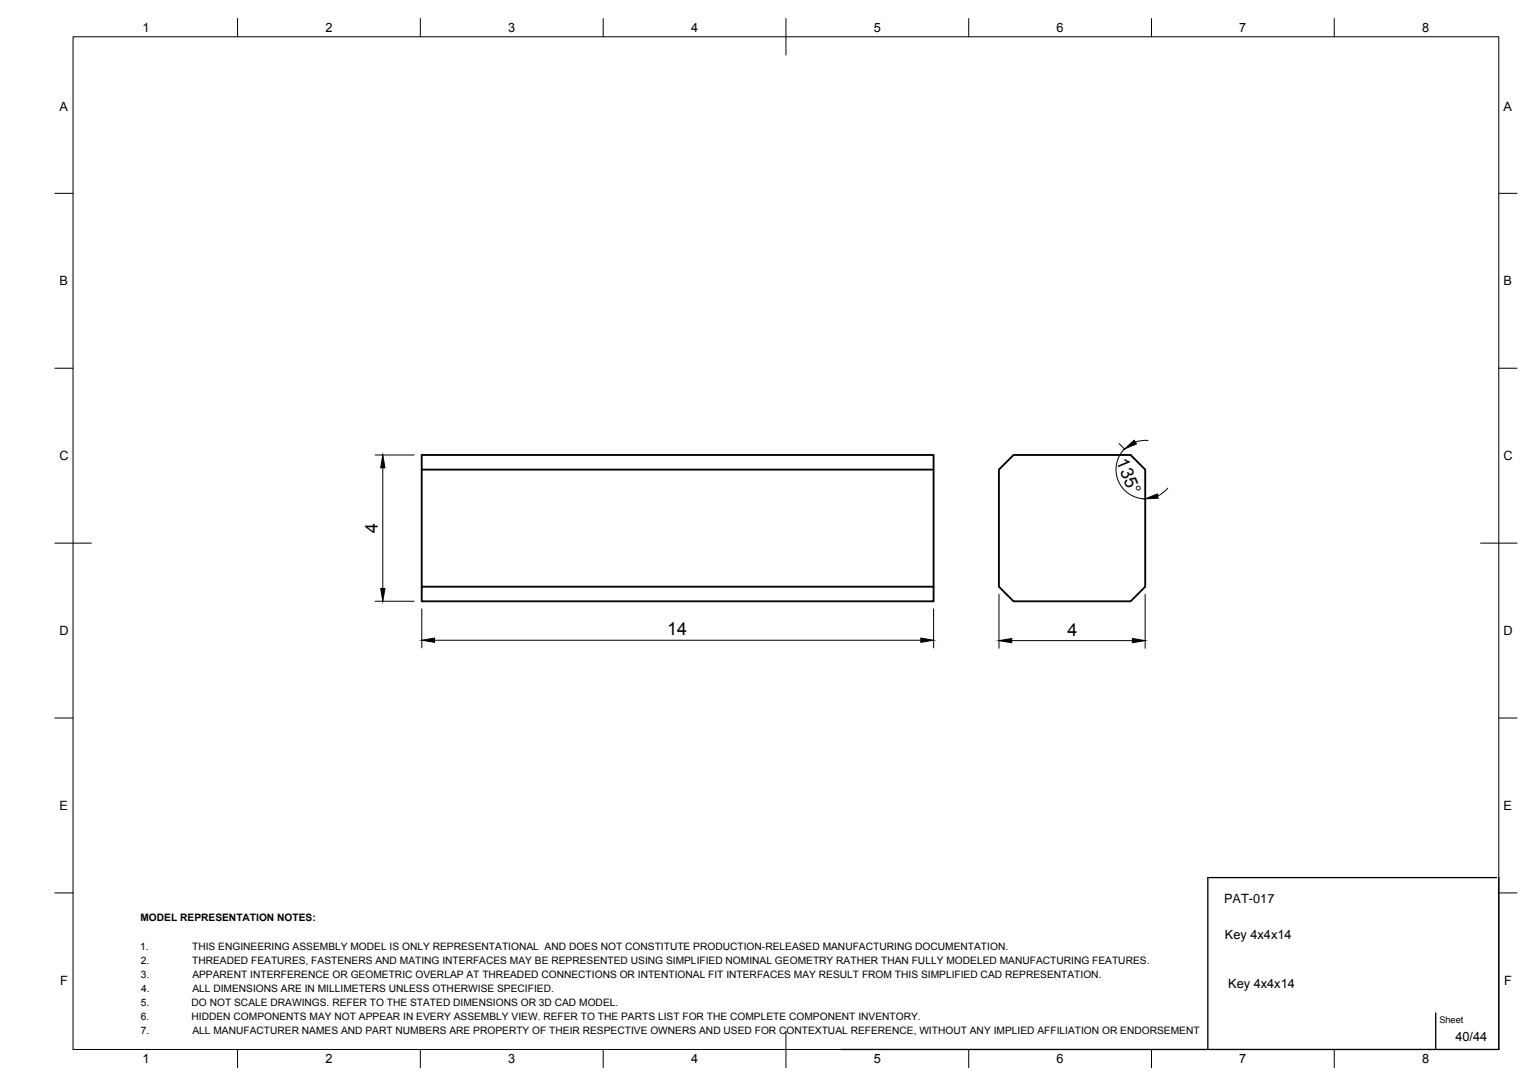
ISO-10303-21;
HEADER;
/* Generated by software containing ST-Developer
 * from STEP Tools, Inc. (www.steptools.com) 
 */

FILE_DESCRIPTION(
/* description */ ('Cam-and-follower valve demonstrator'),
/* implementation_level */ '2;1');

FILE_NAME(
/* name */ 'Key 4x4x14.step',
/* time_stamp */ '2026-10-28T03:25:17-07:00',
/* author */ (''),
/* organization */ (''),
/* preprocessor_version */ 'ST-DEVELOPER v20.2',
/* originating_system */ 'Autodesk Translation Framework v15.17.0.0',
/* authorisation */ '');

FILE_SCHEMA (('AUTOMOTIVE_DESIGN { 1 0 10303 214 3 1 1 }'));
ENDSEC;

DATA;
#10=MECHANICAL_DESIGN_GEOMETRIC_PRESENTATION_REPRESENTATION('',(#450),#12896);
#371=SHAPE_REPRESENTATION_RELATIONSHIP('SRR','None',#13090,#407);
#407=ADVANCED_BREP_SHAPE_REPRESENTATION('',(#491),#12890);
#450=STYLED_ITEM('',(#13330),#491);
#491=MANIFOLD_SOLID_BREP('Body1',#6219);
#1418=FACE_OUTER_BOUND('',#1943,.T.);
#1419=FACE_OUTER_BOUND('',#1944,.T.);
#1420=FACE_OUTER_BOUND('',#1945,.T.);
#1421=FACE_OUTER_BOUND('',#1946,.T.);
#1422=FACE_OUTER_BOUND('',#1947,.T.);
#1423=FACE_OUTER_BOUND('',#1948,.T.);
#1424=FACE_OUTER_BOUND('',#1949,.T.);
#1425=FACE_OUTER_BOUND('',#1950,.T.);
#1426=FACE_OUTER_BOUND('',#1951,.T.);
#1427=FACE_OUTER_BOUND('',#1952,.T.);
#1943=EDGE_LOOP('',(#5425,#5426,#5427,#5428,#5429,#5430,#5431,#5432));
#1944=EDGE_LOOP('',(#5433,#5434,#5435,#5436));
#1945=EDGE_LOOP('',(#5437,#5438,#5439,#5440));
#1946=EDGE_LOOP('',(#5441,#5442,#5443,#5444));
#1947=EDGE_LOOP('',(#5445,#5446,#5447,#5448));
#1948=EDGE_LOOP('',(#5449,#5450,#5451,#5452,#5453,#5454,#5455,#5456));
#1949=EDGE_LOOP('',(#5457,#5458,#5459,#5460));
#1950=EDGE_LOOP('',(#5461,#5462,#5463,#5464));
#1951=EDGE_LOOP('',(#5465,#5466,#5467,#5468));
#1952=EDGE_LOOP('',(#5469,#5470,#5471,#5472));
#2351=LINE('',#12560,#2773);
#2352=LINE('',#12562,#2774);
#2353=LINE('',#12564,#2775);
#2354=LINE('',#12566,#2776);
#2355=LINE('',#12568,#2777);
#2356=LINE('',#12570,#2778);
#2357=LINE('',#12572,#2779);
#2358=LINE('',#12573,#2780);
#2359=LINE('',#12576,#2781);
#2360=LINE('',#12578,#2782);
#2361=LINE('',#12579,#2783);
#2362=LINE('',#12582,#2784);
#2363=LINE('',#12583,#2785);
#2364=LINE('',#12586,#2786);
#2365=LINE('',#12587,#2787);
#2366=LINE('',#12590,#2788);
#2367=LINE('',#12591,#2789);
#2368=LINE('',#12594,#2790);
#2369=LINE('',#12596,#2791);
#2370=LINE('',#12598,#2792);
#2371=LINE('',#12599,#2793);
#2372=LINE('',#12601,#2794);
#2373=LINE('',#12603,#2795);
#2374=LINE('',#12605,#2796);
#2773=VECTOR('',#9092,1.);
#2774=VECTOR('',#9093,1.);
#2775=VECTOR('',#9094,1.);
#2776=VECTOR('',#9095,1.);
#2777=VECTOR('',#9096,1.);
#2778=VECTOR('',#9097,1.);
#2779=VECTOR('',#9098,1.);
#2780=VECTOR('',#9099,1.);
#2781=VECTOR('',#9102,1.);
#2782=VECTOR('',#9103,1.);
#2783=VECTOR('',#9104,1.);
#2784=VECTOR('',#9107,1.);
#2785=VECTOR('',#9108,1.);
#2786=VECTOR('',#9111,1.);
#2787=VECTOR('',#9112,1.);
#2788=VECTOR('',#9115,1.);
#2789=VECTOR('',#9116,1.);
#2790=VECTOR('',#9119,1.);
#2791=VECTOR('',#9120,1.);
#2792=VECTOR('',#9121,1.);
#2793=VECTOR('',#9122,1.);
#2794=VECTOR('',#9125,1.);
#2795=VECTOR('',#9128,1.);
#2796=VECTOR('',#9131,1.);
#3288=VERTEX_POINT('',#12558);
#3289=VERTEX_POINT('',#12559);
#3290=VERTEX_POINT('',#12561);
#3291=VERTEX_POINT('',#12563);
#3292=VERTEX_POINT('',#12565);
#3293=VERTEX_POINT('',#12567);
#3294=VERTEX_POINT('',#12569);
#3295=VERTEX_POINT('',#12571);
#3296=VERTEX_POINT('',#12575);
#3297=VERTEX_POINT('',#12577);
#3298=VERTEX_POINT('',#12581);
#3299=VERTEX_POINT('',#12585);
#3300=VERTEX_POINT('',#12589);
#3301=VERTEX_POINT('',#12593);
#3302=VERTEX_POINT('',#12595);
#3303=VERTEX_POINT('',#12597);
#4009=EDGE_CURVE('',#3288,#3289,#2351,.T.);
#4010=EDGE_CURVE('',#3290,#3288,#2352,.T.);
#4011=EDGE_CURVE('',#3291,#3290,#2353,.T.);
#4012=EDGE_CURVE('',#3292,#3291,#2354,.T.);
#4013=EDGE_CURVE('',#3293,#3292,#2355,.T.);
#4014=EDGE_CURVE('',#3294,#3293,#2356,.T.);
#4015=EDGE_CURVE('',#3295,#3294,#2357,.T.);
#4016=EDGE_CURVE('',#3289,#3295,#2358,.T.);
#4017=EDGE_CURVE('',#3292,#3296,#2359,.T.);
#4018=EDGE_CURVE('',#3296,#3297,#2360,.T.);
#4019=EDGE_CURVE('',#3297,#3293,#2361,.T.);
#4020=EDGE_CURVE('',#3298,#3291,#2362,.T.);
#4021=EDGE_CURVE('',#3298,#3296,#2363,.T.);
#4022=EDGE_CURVE('',#3290,#3299,#2364,.T.);
#4023=EDGE_CURVE('',#3299,#3298,#2365,.T.);
#4024=EDGE_CURVE('',#3300,#3288,#2366,.T.);
#4025=EDGE_CURVE('',#3300,#3299,#2367,.T.);
#4026=EDGE_CURVE('',#3301,#3300,#2368,.T.);
#4027=EDGE_CURVE('',#3302,#3301,#2369,.T.);
#4028=EDGE_CURVE('',#3303,#3302,#2370,.T.);
#4029=EDGE_CURVE('',#3297,#3303,#2371,.T.);
#4030=EDGE_CURVE('',#3289,#3301,#2372,.T.);
#4031=EDGE_CURVE('',#3302,#3295,#2373,.T.);
#4032=EDGE_CURVE('',#3294,#3303,#2374,.T.);
#5425=ORIENTED_EDGE('',*,*,#4009,.F.);
#5426=ORIENTED_EDGE('',*,*,#4010,.F.);
#5427=ORIENTED_EDGE('',*,*,#4011,.F.);
#5428=ORIENTED_EDGE('',*,*,#4012,.F.);
#5429=ORIENTED_EDGE('',*,*,#4013,.F.);
#5430=ORIENTED_EDGE('',*,*,#4014,.F.);
#5431=ORIENTED_EDGE('',*,*,#4015,.F.);
#5432=ORIENTED_EDGE('',*,*,#4016,.F.);
#5433=ORIENTED_EDGE('',*,*,#4013,.T.);
#5434=ORIENTED_EDGE('',*,*,#4017,.T.);
#5435=ORIENTED_EDGE('',*,*,#4018,.T.);
#5436=ORIENTED_EDGE('',*,*,#4019,.T.);
#5437=ORIENTED_EDGE('',*,*,#4012,.T.);
#5438=ORIENTED_EDGE('',*,*,#4020,.F.);
#5439=ORIENTED_EDGE('',*,*,#4021,.T.);
#5440=ORIENTED_EDGE('',*,*,#4017,.F.);
#5441=ORIENTED_EDGE('',*,*,#4011,.T.);
#5442=ORIENTED_EDGE('',*,*,#4022,.T.);
#5443=ORIENTED_EDGE('',*,*,#4023,.T.);
#5444=ORIENTED_EDGE('',*,*,#4020,.T.);
#5445=ORIENTED_EDGE('',*,*,#4010,.T.);
#5446=ORIENTED_EDGE('',*,*,#4024,.F.);
#5447=ORIENTED_EDGE('',*,*,#4025,.T.);
#5448=ORIENTED_EDGE('',*,*,#4022,.F.);
#5449=ORIENTED_EDGE('',*,*,#4018,.F.);
#5450=ORIENTED_EDGE('',*,*,#4021,.F.);
#5451=ORIENTED_EDGE('',*,*,#4023,.F.);
#5452=ORIENTED_EDGE('',*,*,#4025,.F.);
#5453=ORIENTED_EDGE('',*,*,#4026,.F.);
#5454=ORIENTED_EDGE('',*,*,#4027,.F.);
#5455=ORIENTED_EDGE('',*,*,#4028,.F.);
#5456=ORIENTED_EDGE('',*,*,#4029,.F.);
#5457=ORIENTED_EDGE('',*,*,#4009,.T.);
#5458=ORIENTED_EDGE('',*,*,#4030,.T.);
#5459=ORIENTED_EDGE('',*,*,#4026,.T.);
#5460=ORIENTED_EDGE('',*,*,#4024,.T.);
#5461=ORIENTED_EDGE('',*,*,#4016,.T.);
#5462=ORIENTED_EDGE('',*,*,#4031,.F.);
#5463=ORIENTED_EDGE('',*,*,#4027,.T.);
#5464=ORIENTED_EDGE('',*,*,#4030,.F.);
#5465=ORIENTED_EDGE('',*,*,#4015,.T.);
#5466=ORIENTED_EDGE('',*,*,#4032,.T.);
#5467=ORIENTED_EDGE('',*,*,#4028,.T.);
#5468=ORIENTED_EDGE('',*,*,#4031,.T.);
#5469=ORIENTED_EDGE('',*,*,#4014,.T.);
#5470=ORIENTED_EDGE('',*,*,#4019,.F.);
#5471=ORIENTED_EDGE('',*,*,#4029,.T.);
#5472=ORIENTED_EDGE('',*,*,#4032,.F.);
#5778=PLANE('',#7282);
#5779=PLANE('',#7283);
#5780=PLANE('',#7284);
#5781=PLANE('',#7285);
#5782=PLANE('',#7286);
#5783=PLANE('',#7287);
#5784=PLANE('',#7288);
#5785=PLANE('',#7289);
#5786=PLANE('',#7290);
#5787=PLANE('',#7291);
#6134=ADVANCED_FACE('',(#1418),#5778,.T.);
#6135=ADVANCED_FACE('',(#1419),#5779,.T.);
#6136=ADVANCED_FACE('',(#1420),#5780,.T.);
#6137=ADVANCED_FACE('',(#1421),#5781,.T.);
#6138=ADVANCED_FACE('',(#1422),#5782,.T.);
#6139=ADVANCED_FACE('',(#1423),#5783,.F.);
#6140=ADVANCED_FACE('',(#1424),#5784,.T.);
#6141=ADVANCED_FACE('',(#1425),#5785,.T.);
#6142=ADVANCED_FACE('',(#1426),#5786,.T.);
#6143=ADVANCED_FACE('',(#1427),#5787,.F.);
#6219=CLOSED_SHELL('',(#6134,#6135,#6136,#6137,#6138,#6139,#6140,#6141,
#6142,#6143));
#7281=AXIS2_PLACEMENT_3D('',#12556,#9088,#9089);
#7282=AXIS2_PLACEMENT_3D('',#12557,#9090,#9091);
#7283=AXIS2_PLACEMENT_3D('',#12574,#9100,#9101);
#7284=AXIS2_PLACEMENT_3D('',#12580,#9105,#9106);
#7285=AXIS2_PLACEMENT_3D('',#12584,#9109,#9110);
#7286=AXIS2_PLACEMENT_3D('',#12588,#9113,#9114);
#7287=AXIS2_PLACEMENT_3D('',#12592,#9117,#9118);
#7288=AXIS2_PLACEMENT_3D('',#12600,#9123,#9124);
#7289=AXIS2_PLACEMENT_3D('',#12602,#9126,#9127);
#7290=AXIS2_PLACEMENT_3D('',#12604,#9129,#9130);
#7291=AXIS2_PLACEMENT_3D('',#12606,#9132,#9133);
#9088=DIRECTION('axis',(0.,0.,1.));
#9089=DIRECTION('refdir',(1.,0.,0.));
#9090=DIRECTION('center_axis',(1.,0.,0.));
#9091=DIRECTION('ref_axis',(0.,0.,-1.));
#9092=DIRECTION('',(0.,0.707106781186547,-0.707106781186548));
#9093=DIRECTION('',(0.,1.,0.));
#9094=DIRECTION('',(0.,0.707106781186547,0.707106781186548));
#9095=DIRECTION('',(0.,0.,1.));
#9096=DIRECTION('',(0.,-0.707106781186548,0.707106781186548));
#9097=DIRECTION('',(0.,-1.,0.));
#9098=DIRECTION('',(0.,-0.707106781186548,-0.707106781186548));
#9099=DIRECTION('',(0.,0.,-1.));
#9100=DIRECTION('center_axis',(0.,-0.707106781186548,-0.707106781186548));
#9101=DIRECTION('ref_axis',(-1.,0.,0.));
#9102=DIRECTION('',(-1.,0.,0.));
#9103=DIRECTION('',(0.,0.707106781186548,-0.707106781186548));
#9104=DIRECTION('',(1.,0.,0.));
#9105=DIRECTION('center_axis',(0.,-1.,0.));
#9106=DIRECTION('ref_axis',(1.,0.,0.));
#9107=DIRECTION('',(1.,0.,0.));
#9108=DIRECTION('',(0.,0.,-1.));
#9109=DIRECTION('center_axis',(0.,-0.707106781186548,0.707106781186547));
#9110=DIRECTION('ref_axis',(1.,0.,0.));
#9111=DIRECTION('',(-1.,0.,0.));
#9112=DIRECTION('',(0.,-0.707106781186547,-0.707106781186548));
#9113=DIRECTION('center_axis',(0.,0.,1.));
#9114=DIRECTION('ref_axis',(1.,0.,0.));
#9115=DIRECTION('',(1.,0.,0.));
#9116=DIRECTION('',(0.,-1.,0.));
#9117=DIRECTION('center_axis',(1.,0.,0.));
#9118=DIRECTION('ref_axis',(0.,0.,-1.));
#9119=DIRECTION('',(0.,-0.707106781186547,0.707106781186548));
#9120=DIRECTION('',(0.,0.,1.));
#9121=DIRECTION('',(0.,0.707106781186548,0.707106781186548));
#9122=DIRECTION('',(0.,1.,0.));
#9123=DIRECTION('center_axis',(0.,0.707106781186548,0.707106781186547));
#9124=DIRECTION('ref_axis',(1.,0.,0.));
#9125=DIRECTION('',(-1.,0.,0.));
#9126=DIRECTION('center_axis',(0.,1.,0.));
#9127=DIRECTION('ref_axis',(-1.,0.,0.));
#9128=DIRECTION('',(1.,0.,0.));
#9129=DIRECTION('center_axis',(0.,0.707106781186548,-0.707106781186548));
#9130=DIRECTION('ref_axis',(-1.,0.,0.));
#9131=DIRECTION('',(-1.,0.,0.));
#9132=DIRECTION('center_axis',(0.,0.,1.));
#9133=DIRECTION('ref_axis',(1.,0.,0.));
#12556=CARTESIAN_POINT('',(0.,0.,0.));
#12557=CARTESIAN_POINT('Origin',(0.7,0.,0.25));
#12558=CARTESIAN_POINT('',(0.7,0.16,0.4));
#12559=CARTESIAN_POINT('',(0.7,0.2,0.36));
#12560=CARTESIAN_POINT('',(0.7,0.1675,0.3925));
#12561=CARTESIAN_POINT('',(0.7,-0.16,0.4));
#12562=CARTESIAN_POINT('',(0.7,0.,0.4));
#12563=CARTESIAN_POINT('',(0.7,-0.2,0.36));
#12564=CARTESIAN_POINT('',(0.7,-0.1675,0.3925));
#12565=CARTESIAN_POINT('',(0.7,-0.2,0.04));
#12566=CARTESIAN_POINT('',(0.7,-0.2,0.125));
#12567=CARTESIAN_POINT('',(0.7,-0.16,0.));
#12568=CARTESIAN_POINT('',(0.7,-0.1925,0.0325));
#12569=CARTESIAN_POINT('',(0.7,0.16,0.));
#12570=CARTESIAN_POINT('',(0.7,0.,0.));
#12571=CARTESIAN_POINT('',(0.7,0.2,0.04));
#12572=CARTESIAN_POINT('',(0.7,0.1925,0.0325));
#12573=CARTESIAN_POINT('',(0.7,0.2,0.125));
#12574=CARTESIAN_POINT('Origin',(-0.4,-0.18,0.02));
#12575=CARTESIAN_POINT('',(-0.7,-0.2,0.04));
#12576=CARTESIAN_POINT('',(-0.4,-0.2,0.04));
#12577=CARTESIAN_POINT('',(-0.7,-0.16,0.));
#12578=CARTESIAN_POINT('',(-0.7,-0.1925,0.0325));
#12579=CARTESIAN_POINT('',(-0.4,-0.16,0.));
#12580=CARTESIAN_POINT('Origin',(-0.8,-0.2,0.));
#12581=CARTESIAN_POINT('',(-0.7,-0.2,0.36));
#12582=CARTESIAN_POINT('',(-0.4,-0.2,0.36));
#12583=CARTESIAN_POINT('',(-0.7,-0.2,0.125));
#12584=CARTESIAN_POINT('Origin',(-0.4,-0.18,0.38));
#12585=CARTESIAN_POINT('',(-0.7,-0.16,0.4));
#12586=CARTESIAN_POINT('',(-0.4,-0.16,0.4));
#12587=CARTESIAN_POINT('',(-0.7,-0.1675,0.3925));
#12588=CARTESIAN_POINT('Origin',(0.,0.,0.4));
#12589=CARTESIAN_POINT('',(-0.7,0.16,0.4));
#12590=CARTESIAN_POINT('',(0.4,0.16,0.4));
#12591=CARTESIAN_POINT('',(-0.7,0.,0.4));
#12592=CARTESIAN_POINT('Origin',(-0.7,0.,0.25));
#12593=CARTESIAN_POINT('',(-0.7,0.2,0.36));
#12594=CARTESIAN_POINT('',(-0.7,0.1675,0.3925));
#12595=CARTESIAN_POINT('',(-0.7,0.2,0.04));
#12596=CARTESIAN_POINT('',(-0.7,0.2,0.125));
#12597=CARTESIAN_POINT('',(-0.7,0.16,0.));
#12598=CARTESIAN_POINT('',(-0.7,0.1925,0.0325));
#12599=CARTESIAN_POINT('',(-0.7,0.,0.));
#12600=CARTESIAN_POINT('Origin',(0.4,0.18,0.38));
#12601=CARTESIAN_POINT('',(0.4,0.2,0.36));
#12602=CARTESIAN_POINT('Origin',(0.8,0.2,0.));
#12603=CARTESIAN_POINT('',(0.4,0.2,0.04));
#12604=CARTESIAN_POINT('Origin',(0.4,0.18,0.02));
#12605=CARTESIAN_POINT('',(0.4,0.16,0.));
#12606=CARTESIAN_POINT('Origin',(0.,0.,0.));
#12847=UNCERTAINTY_MEASURE_WITH_UNIT(LENGTH_MEASURE(0.001),#12897,
'DISTANCE_ACCURACY_VALUE',
'Maximum model space distance between geometric entities at asserted c
onnectivities');
#12853=UNCERTAINTY_MEASURE_WITH_UNIT(LENGTH_MEASURE(0.001),#12897,
'DISTANCE_ACCURACY_VALUE',
'Maximum model space distance between geometric entities at asserted c
onnectivities');
#12890=(
GEOMETRIC_REPRESENTATION_CONTEXT(3)
GLOBAL_UNCERTAINTY_ASSIGNED_CONTEXT((#12847))
GLOBAL_UNIT_ASSIGNED_CONTEXT((#12897,#12899,#12900))
REPRESENTATION_CONTEXT('','3D')
);
#12896=(
GEOMETRIC_REPRESENTATION_CONTEXT(3)
GLOBAL_UNCERTAINTY_ASSIGNED_CONTEXT((#12853))
GLOBAL_UNIT_ASSIGNED_CONTEXT((#12897,#12899,#12900))
REPRESENTATION_CONTEXT('','3D')
);
#12897=(
LENGTH_UNIT()
NAMED_UNIT(*)
SI_UNIT(.CENTI.,.METRE.)
);
#12899=(
NAMED_UNIT(*)
PLANE_ANGLE_UNIT()
SI_UNIT($,.RADIAN.)
);
#12900=(
NAMED_UNIT(*)
SI_UNIT($,.STERADIAN.)
SOLID_ANGLE_UNIT()
);
#12937=SHAPE_DEFINITION_REPRESENTATION(#12986,#13090);
#12986=PRODUCT_DEFINITION_SHAPE('',$,#13133);
#13090=SHAPE_REPRESENTATION('',(#7281),#12890);
#13096=PRODUCT_DEFINITION_CONTEXT('part definition',#13224,'design');
#13133=PRODUCT_DEFINITION('Key 4x4x14','Key 4x4x14',#13175,#13096);
#13175=PRODUCT_DEFINITION_FORMATION('',$,#13262);
#13224=APPLICATION_CONTEXT(
'Core Data for Automotive Mechanical Design Process');
#13225=PRODUCT_CONTEXT('part definition',#13224,'mechanical');
#13262=PRODUCT('Key 4x4x14','Key 4x4x14','Key 4x4x14',(#13225));
#13324=COLOUR_RGB('Grey',0.48,0.52,0.57);
#13325=FILL_AREA_STYLE_COLOUR('',#13324);
#13326=FILL_AREA_STYLE('',(#13325));
#13327=SURFACE_STYLE_FILL_AREA(#13326);
#13328=SURFACE_SIDE_STYLE('',(#13327));
#13329=SURFACE_STYLE_USAGE(.BOTH.,#13328);
#13330=PRESENTATION_STYLE_ASSIGNMENT((#13329));
ENDSEC;
END-ISO-10303-21;
